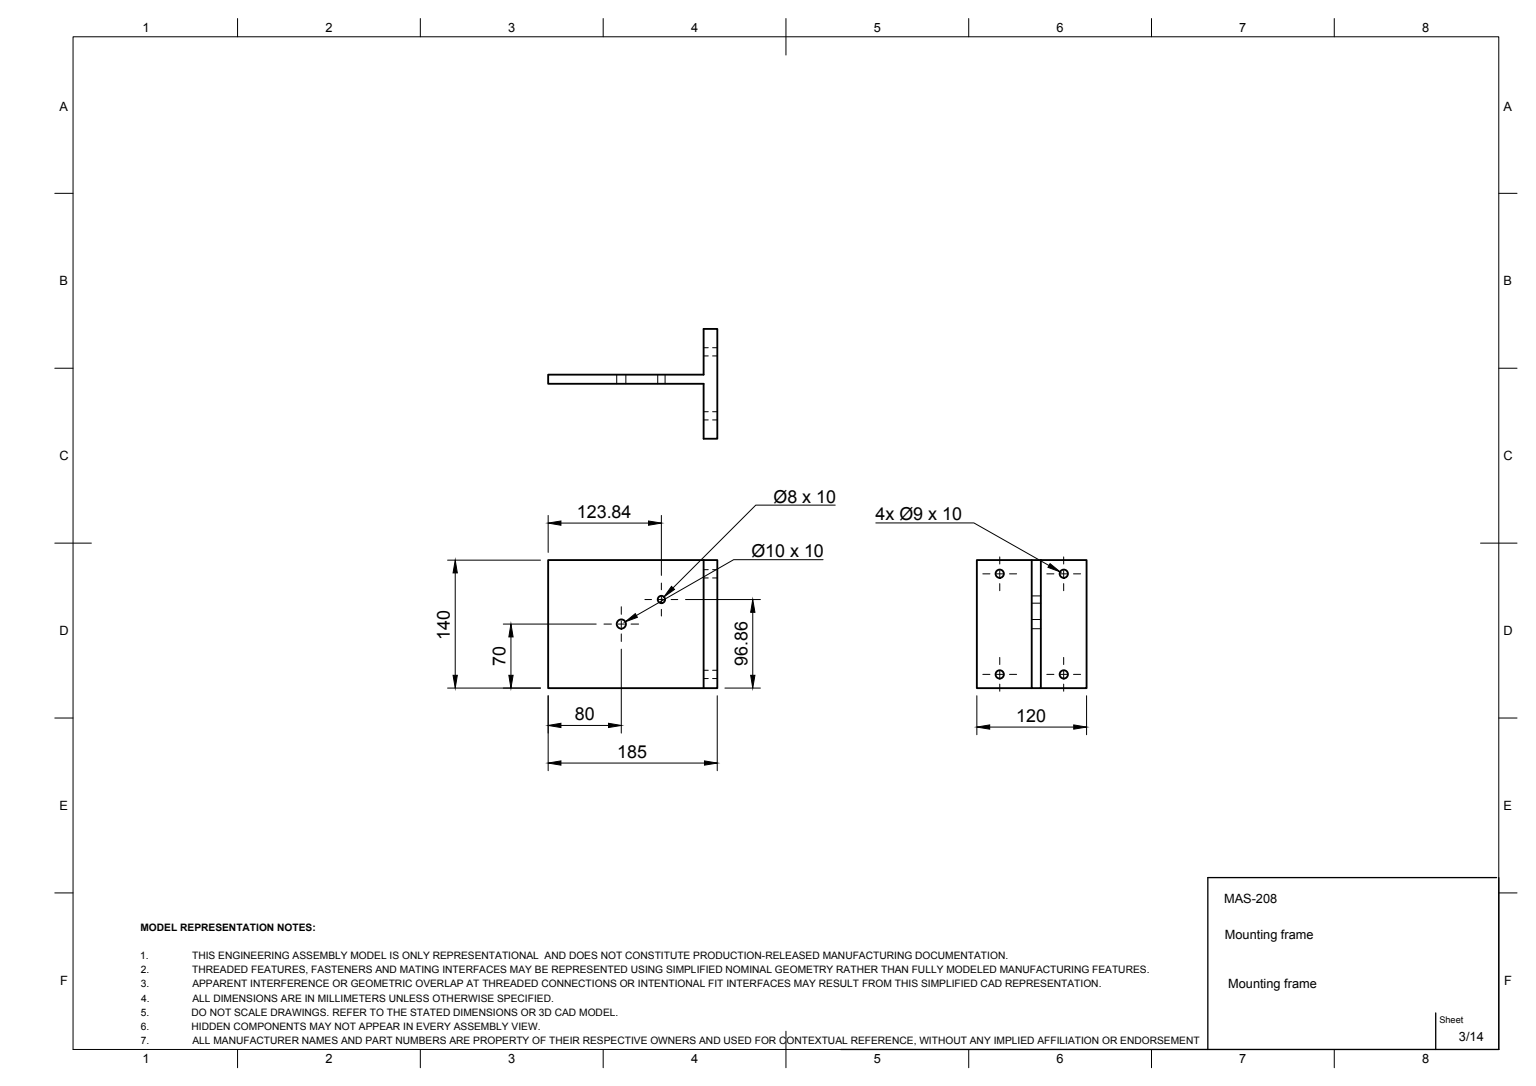
ISO-10303-21;
HEADER;
/* Generated by software containing ST-Developer
 * from STEP Tools, Inc. (www.steptools.com) 
 */

FILE_DESCRIPTION(
/* description */ ('Independent vertical20-tooth ratchet advance with repeated integral-c
ounterweight gravity pawls, swinging drive lever, bronze sleeves and f
ully retained axle stacks.18degpertooth. Native revolutes; geometric c
ycle checking rather than automatic contact/rolling dynamics. Gravity 
closing checked from actual pawl center of mass. Backplate/foot suppor
ts unit. Fits, torque, holding force, wear and life unassigned.'),
/* implementation_level */ '2;1');

FILE_NAME(
/* name */ 'Mounting frame.step',
/* time_stamp */ '2026-11-09T06:25:53-08:00',
/* author */ (''),
/* organization */ (''),
/* preprocessor_version */ 'ST-DEVELOPER v20.2',
/* originating_system */ 'Autodesk Translation Framework v15.17.0.0',
/* authorisation */ '');

FILE_SCHEMA (('AUTOMOTIVE_DESIGN { 1 0 10303 214 3 1 1 }'));
ENDSEC;

DATA;
#10=MECHANICAL_DESIGN_GEOMETRIC_PRESENTATION_REPRESENTATION('',(#123),#4643);
#95=SHAPE_REPRESENTATION_RELATIONSHIP('SRR','None',#4700,#109);
#109=ADVANCED_BREP_SHAPE_REPRESENTATION('',(#137),#4629);
#123=STYLED_ITEM('',(#4779),#137);
#137=MANIFOLD_SOLID_BREP('Body1',#2659);
#151=FACE_BOUND('',#460,.T.);
#152=FACE_BOUND('',#461,.T.);
#153=FACE_BOUND('',#463,.T.);
#154=FACE_BOUND('',#464,.T.);
#155=FACE_BOUND('',#466,.T.);
#156=FACE_BOUND('',#467,.T.);
#157=FACE_BOUND('',#468,.T.);
#158=FACE_BOUND('',#469,.T.);
#159=FACE_BOUND('',#476,.T.);
#160=FACE_BOUND('',#477,.T.);
#161=FACE_BOUND('',#479,.T.);
#162=FACE_BOUND('',#480,.T.);
#192=PLANE('',#2848);
#193=PLANE('',#2849);
#194=PLANE('',#2850);
#195=PLANE('',#2851);
#196=PLANE('',#2852);
#197=PLANE('',#2853);
#198=PLANE('',#2854);
#199=PLANE('',#2855);
#200=PLANE('',#2856);
#201=PLANE('',#2857);
#304=FACE_OUTER_BOUND('',#453,.T.);
#305=FACE_OUTER_BOUND('',#454,.T.);
#306=FACE_OUTER_BOUND('',#455,.T.);
#307=FACE_OUTER_BOUND('',#456,.T.);
#308=FACE_OUTER_BOUND('',#457,.T.);
#309=FACE_OUTER_BOUND('',#458,.T.);
#310=FACE_OUTER_BOUND('',#459,.T.);
#311=FACE_OUTER_BOUND('',#462,.T.);
#312=FACE_OUTER_BOUND('',#465,.T.);
#313=FACE_OUTER_BOUND('',#470,.T.);
#314=FACE_OUTER_BOUND('',#471,.T.);
#315=FACE_OUTER_BOUND('',#472,.T.);
#316=FACE_OUTER_BOUND('',#473,.T.);
#317=FACE_OUTER_BOUND('',#474,.T.);
#318=FACE_OUTER_BOUND('',#475,.T.);
#319=FACE_OUTER_BOUND('',#478,.T.);
#453=EDGE_LOOP('',(#1801,#1802,#1803,#1804));
#454=EDGE_LOOP('',(#1805,#1806,#1807,#1808));
#455=EDGE_LOOP('',(#1809,#1810,#1811,#1812));
#456=EDGE_LOOP('',(#1813,#1814,#1815,#1816));
#457=EDGE_LOOP('',(#1817,#1818,#1819,#1820));
#458=EDGE_LOOP('',(#1821,#1822,#1823,#1824));
#459=EDGE_LOOP('',(#1825,#1826,#1827,#1828));
#460=EDGE_LOOP('',(#1829));
#461=EDGE_LOOP('',(#1830));
#462=EDGE_LOOP('',(#1831,#1832,#1833,#1834));
#463=EDGE_LOOP('',(#1835));
#464=EDGE_LOOP('',(#1836));
#465=EDGE_LOOP('',(#1837,#1838,#1839,#1840));
#466=EDGE_LOOP('',(#1841));
#467=EDGE_LOOP('',(#1842));
#468=EDGE_LOOP('',(#1843));
#469=EDGE_LOOP('',(#1844));
#470=EDGE_LOOP('',(#1845,#1846,#1847,#1848));
#471=EDGE_LOOP('',(#1849,#1850,#1851,#1852));
#472=EDGE_LOOP('',(#1853,#1854,#1855,#1856));
#473=EDGE_LOOP('',(#1857,#1858,#1859,#1860,#1861,#1862,#1863,#1864));
#474=EDGE_LOOP('',(#1865,#1866,#1867,#1868,#1869,#1870,#1871,#1872));
#475=EDGE_LOOP('',(#1873,#1874,#1875,#1876));
#476=EDGE_LOOP('',(#1877));
#477=EDGE_LOOP('',(#1878));
#478=EDGE_LOOP('',(#1879,#1880,#1881,#1882));
#479=EDGE_LOOP('',(#1883));
#480=EDGE_LOOP('',(#1884));
#643=LINE('',#3873,#905);
#644=LINE('',#3879,#906);
#645=LINE('',#3885,#907);
#646=LINE('',#3891,#908);
#647=LINE('',#3897,#909);
#648=LINE('',#3903,#910);
#649=LINE('',#3908,#911);
#650=LINE('',#3910,#912);
#651=LINE('',#3912,#913);
#652=LINE('',#3913,#914);
#653=LINE('',#3917,#915);
#654=LINE('',#3919,#916);
#655=LINE('',#3921,#917);
#656=LINE('',#3922,#918);
#657=LINE('',#3926,#919);
#658=LINE('',#3928,#920);
#659=LINE('',#3930,#921);
#660=LINE('',#3931,#922);
#661=LINE('',#3933,#923);
#662=LINE('',#3934,#924);
#663=LINE('',#3936,#925);
#664=LINE('',#3937,#926);
#665=LINE('',#3941,#927);
#666=LINE('',#3943,#928);
#667=LINE('',#3945,#929);
#668=LINE('',#3946,#930);
#669=LINE('',#3948,#931);
#670=LINE('',#3949,#932);
#671=LINE('',#3951,#933);
#672=LINE('',#3952,#934);
#905=VECTOR('',#3095,4.);
#906=VECTOR('',#3102,5.);
#907=VECTOR('',#3109,4.5);
#908=VECTOR('',#3116,4.5);
#909=VECTOR('',#3123,4.5);
#910=VECTOR('',#3130,4.5);
#911=VECTOR('',#3135,10.);
#912=VECTOR('',#3136,10.);
#913=VECTOR('',#3137,10.);
#914=VECTOR('',#3138,10.);
#915=VECTOR('',#3141,10.);
#916=VECTOR('',#3142,10.);
#917=VECTOR('',#3143,10.);
#918=VECTOR('',#3144,10.);
#919=VECTOR('',#3147,10.);
#920=VECTOR('',#3148,10.);
#921=VECTOR('',#3149,10.);
#922=VECTOR('',#3150,10.);
#923=VECTOR('',#3153,10.);
#924=VECTOR('',#3154,10.);
#925=VECTOR('',#3157,10.);
#926=VECTOR('',#3158,10.);
#927=VECTOR('',#3161,10.);
#928=VECTOR('',#3162,10.);
#929=VECTOR('',#3163,10.);
#930=VECTOR('',#3164,10.);
#931=VECTOR('',#3167,10.);
#932=VECTOR('',#3168,10.);
#933=VECTOR('',#3171,10.);
#934=VECTOR('',#3172,10.);
#1167=CIRCLE('',#2831,4.);
#1168=CIRCLE('',#2832,4.);
#1169=CIRCLE('',#2834,5.);
#1170=CIRCLE('',#2835,5.);
#1171=CIRCLE('',#2837,4.5);
#1172=CIRCLE('',#2838,4.5);
#1173=CIRCLE('',#2840,4.5);
#1174=CIRCLE('',#2841,4.5);
#1175=CIRCLE('',#2843,4.5);
#1176=CIRCLE('',#2844,4.5);
#1177=CIRCLE('',#2846,4.5);
#1178=CIRCLE('',#2847,4.5);
#1241=VERTEX_POINT('',#3870);
#1242=VERTEX_POINT('',#3872);
#1243=VERTEX_POINT('',#3876);
#1244=VERTEX_POINT('',#3878);
#1245=VERTEX_POINT('',#3882);
#1246=VERTEX_POINT('',#3884);
#1247=VERTEX_POINT('',#3888);
#1248=VERTEX_POINT('',#3890);
#1249=VERTEX_POINT('',#3894);
#1250=VERTEX_POINT('',#3896);
#1251=VERTEX_POINT('',#3900);
#1252=VERTEX_POINT('',#3902);
#1253=VERTEX_POINT('',#3906);
#1254=VERTEX_POINT('',#3907);
#1255=VERTEX_POINT('',#3909);
#1256=VERTEX_POINT('',#3911);
#1257=VERTEX_POINT('',#3915);
#1258=VERTEX_POINT('',#3916);
#1259=VERTEX_POINT('',#3918);
#1260=VERTEX_POINT('',#3920);
#1261=VERTEX_POINT('',#3924);
#1262=VERTEX_POINT('',#3925);
#1263=VERTEX_POINT('',#3927);
#1264=VERTEX_POINT('',#3929);
#1265=VERTEX_POINT('',#3939);
#1266=VERTEX_POINT('',#3940);
#1267=VERTEX_POINT('',#3942);
#1268=VERTEX_POINT('',#3944);
#1465=EDGE_CURVE('',#1241,#1241,#1167,.T.);
#1466=EDGE_CURVE('',#1241,#1242,#643,.T.);
#1467=EDGE_CURVE('',#1242,#1242,#1168,.T.);
#1468=EDGE_CURVE('',#1243,#1243,#1169,.T.);
#1469=EDGE_CURVE('',#1243,#1244,#644,.T.);
#1470=EDGE_CURVE('',#1244,#1244,#1170,.T.);
#1471=EDGE_CURVE('',#1245,#1245,#1171,.F.);
#1472=EDGE_CURVE('',#1245,#1246,#645,.T.);
#1473=EDGE_CURVE('',#1246,#1246,#1172,.T.);
#1474=EDGE_CURVE('',#1247,#1247,#1173,.F.);
#1475=EDGE_CURVE('',#1247,#1248,#646,.T.);
#1476=EDGE_CURVE('',#1248,#1248,#1174,.T.);
#1477=EDGE_CURVE('',#1249,#1249,#1175,.F.);
#1478=EDGE_CURVE('',#1249,#1250,#647,.T.);
#1479=EDGE_CURVE('',#1250,#1250,#1176,.T.);
#1480=EDGE_CURVE('',#1251,#1251,#1177,.F.);
#1481=EDGE_CURVE('',#1251,#1252,#648,.T.);
#1482=EDGE_CURVE('',#1252,#1252,#1178,.T.);
#1483=EDGE_CURVE('',#1253,#1254,#649,.T.);
#1484=EDGE_CURVE('',#1255,#1254,#650,.T.);
#1485=EDGE_CURVE('',#1255,#1256,#651,.T.);
#1486=EDGE_CURVE('',#1256,#1253,#652,.T.);
#1487=EDGE_CURVE('',#1257,#1258,#653,.T.);
#1488=EDGE_CURVE('',#1257,#1259,#654,.T.);
#1489=EDGE_CURVE('',#1260,#1259,#655,.T.);
#1490=EDGE_CURVE('',#1258,#1260,#656,.T.);
#1491=EDGE_CURVE('',#1261,#1262,#657,.T.);
#1492=EDGE_CURVE('',#1262,#1263,#658,.T.);
#1493=EDGE_CURVE('',#1264,#1263,#659,.F.);
#1494=EDGE_CURVE('',#1261,#1264,#660,.F.);
#1495=EDGE_CURVE('',#1259,#1264,#661,.T.);
#1496=EDGE_CURVE('',#1263,#1260,#662,.T.);
#1497=EDGE_CURVE('',#1256,#1261,#663,.T.);
#1498=EDGE_CURVE('',#1262,#1255,#664,.T.);
#1499=EDGE_CURVE('',#1265,#1266,#665,.F.);
#1500=EDGE_CURVE('',#1266,#1267,#666,.T.);
#1501=EDGE_CURVE('',#1268,#1267,#667,.F.);
#1502=EDGE_CURVE('',#1265,#1268,#668,.F.);
#1503=EDGE_CURVE('',#1254,#1265,#669,.T.);
#1504=EDGE_CURVE('',#1258,#1268,#670,.T.);
#1505=EDGE_CURVE('',#1266,#1253,#671,.T.);
#1506=EDGE_CURVE('',#1267,#1257,#672,.T.);
#1801=ORIENTED_EDGE('',*,*,#1465,.F.);
#1802=ORIENTED_EDGE('',*,*,#1466,.T.);
#1803=ORIENTED_EDGE('',*,*,#1467,.F.);
#1804=ORIENTED_EDGE('',*,*,#1466,.F.);
#1805=ORIENTED_EDGE('',*,*,#1468,.F.);
#1806=ORIENTED_EDGE('',*,*,#1469,.T.);
#1807=ORIENTED_EDGE('',*,*,#1470,.F.);
#1808=ORIENTED_EDGE('',*,*,#1469,.F.);
#1809=ORIENTED_EDGE('',*,*,#1471,.F.);
#1810=ORIENTED_EDGE('',*,*,#1472,.T.);
#1811=ORIENTED_EDGE('',*,*,#1473,.F.);
#1812=ORIENTED_EDGE('',*,*,#1472,.F.);
#1813=ORIENTED_EDGE('',*,*,#1474,.F.);
#1814=ORIENTED_EDGE('',*,*,#1475,.T.);
#1815=ORIENTED_EDGE('',*,*,#1476,.F.);
#1816=ORIENTED_EDGE('',*,*,#1475,.F.);
#1817=ORIENTED_EDGE('',*,*,#1477,.F.);
#1818=ORIENTED_EDGE('',*,*,#1478,.T.);
#1819=ORIENTED_EDGE('',*,*,#1479,.F.);
#1820=ORIENTED_EDGE('',*,*,#1478,.F.);
#1821=ORIENTED_EDGE('',*,*,#1480,.F.);
#1822=ORIENTED_EDGE('',*,*,#1481,.T.);
#1823=ORIENTED_EDGE('',*,*,#1482,.F.);
#1824=ORIENTED_EDGE('',*,*,#1481,.F.);
#1825=ORIENTED_EDGE('',*,*,#1483,.T.);
#1826=ORIENTED_EDGE('',*,*,#1484,.F.);
#1827=ORIENTED_EDGE('',*,*,#1485,.T.);
#1828=ORIENTED_EDGE('',*,*,#1486,.T.);
#1829=ORIENTED_EDGE('',*,*,#1473,.T.);
#1830=ORIENTED_EDGE('',*,*,#1476,.T.);
#1831=ORIENTED_EDGE('',*,*,#1487,.F.);
#1832=ORIENTED_EDGE('',*,*,#1488,.T.);
#1833=ORIENTED_EDGE('',*,*,#1489,.F.);
#1834=ORIENTED_EDGE('',*,*,#1490,.F.);
#1835=ORIENTED_EDGE('',*,*,#1479,.T.);
#1836=ORIENTED_EDGE('',*,*,#1482,.T.);
#1837=ORIENTED_EDGE('',*,*,#1491,.T.);
#1838=ORIENTED_EDGE('',*,*,#1492,.T.);
#1839=ORIENTED_EDGE('',*,*,#1493,.F.);
#1840=ORIENTED_EDGE('',*,*,#1494,.F.);
#1841=ORIENTED_EDGE('',*,*,#1471,.T.);
#1842=ORIENTED_EDGE('',*,*,#1474,.T.);
#1843=ORIENTED_EDGE('',*,*,#1477,.T.);
#1844=ORIENTED_EDGE('',*,*,#1480,.T.);
#1845=ORIENTED_EDGE('',*,*,#1495,.T.);
#1846=ORIENTED_EDGE('',*,*,#1493,.T.);
#1847=ORIENTED_EDGE('',*,*,#1496,.T.);
#1848=ORIENTED_EDGE('',*,*,#1489,.T.);
#1849=ORIENTED_EDGE('',*,*,#1497,.F.);
#1850=ORIENTED_EDGE('',*,*,#1485,.F.);
#1851=ORIENTED_EDGE('',*,*,#1498,.F.);
#1852=ORIENTED_EDGE('',*,*,#1491,.F.);
#1853=ORIENTED_EDGE('',*,*,#1499,.T.);
#1854=ORIENTED_EDGE('',*,*,#1500,.T.);
#1855=ORIENTED_EDGE('',*,*,#1501,.F.);
#1856=ORIENTED_EDGE('',*,*,#1502,.F.);
#1857=ORIENTED_EDGE('',*,*,#1503,.T.);
#1858=ORIENTED_EDGE('',*,*,#1502,.T.);
#1859=ORIENTED_EDGE('',*,*,#1504,.F.);
#1860=ORIENTED_EDGE('',*,*,#1490,.T.);
#1861=ORIENTED_EDGE('',*,*,#1496,.F.);
#1862=ORIENTED_EDGE('',*,*,#1492,.F.);
#1863=ORIENTED_EDGE('',*,*,#1498,.T.);
#1864=ORIENTED_EDGE('',*,*,#1484,.T.);
#1865=ORIENTED_EDGE('',*,*,#1505,.T.);
#1866=ORIENTED_EDGE('',*,*,#1486,.F.);
#1867=ORIENTED_EDGE('',*,*,#1497,.T.);
#1868=ORIENTED_EDGE('',*,*,#1494,.T.);
#1869=ORIENTED_EDGE('',*,*,#1495,.F.);
#1870=ORIENTED_EDGE('',*,*,#1488,.F.);
#1871=ORIENTED_EDGE('',*,*,#1506,.F.);
#1872=ORIENTED_EDGE('',*,*,#1500,.F.);
#1873=ORIENTED_EDGE('',*,*,#1506,.T.);
#1874=ORIENTED_EDGE('',*,*,#1487,.T.);
#1875=ORIENTED_EDGE('',*,*,#1504,.T.);
#1876=ORIENTED_EDGE('',*,*,#1501,.T.);
#1877=ORIENTED_EDGE('',*,*,#1465,.T.);
#1878=ORIENTED_EDGE('',*,*,#1468,.T.);
#1879=ORIENTED_EDGE('',*,*,#1505,.F.);
#1880=ORIENTED_EDGE('',*,*,#1499,.F.);
#1881=ORIENTED_EDGE('',*,*,#1503,.F.);
#1882=ORIENTED_EDGE('',*,*,#1483,.F.);
#1883=ORIENTED_EDGE('',*,*,#1467,.T.);
#1884=ORIENTED_EDGE('',*,*,#1470,.T.);
#2473=CYLINDRICAL_SURFACE('',#2830,4.);
#2474=CYLINDRICAL_SURFACE('',#2833,5.);
#2475=CYLINDRICAL_SURFACE('',#2836,4.5);
#2476=CYLINDRICAL_SURFACE('',#2839,4.5);
#2477=CYLINDRICAL_SURFACE('',#2842,4.5);
#2478=CYLINDRICAL_SURFACE('',#2845,4.5);
#2510=ADVANCED_FACE('',(#304),#2473,.F.);
#2511=ADVANCED_FACE('',(#305),#2474,.F.);
#2512=ADVANCED_FACE('',(#306),#2475,.F.);
#2513=ADVANCED_FACE('',(#307),#2476,.F.);
#2514=ADVANCED_FACE('',(#308),#2477,.F.);
#2515=ADVANCED_FACE('',(#309),#2478,.F.);
#2516=ADVANCED_FACE('',(#310,#151,#152),#192,.T.);
#2517=ADVANCED_FACE('',(#311,#153,#154),#193,.T.);
#2518=ADVANCED_FACE('',(#312,#155,#156,#157,#158),#194,.T.);
#2519=ADVANCED_FACE('',(#313),#195,.T.);
#2520=ADVANCED_FACE('',(#314),#196,.F.);
#2521=ADVANCED_FACE('',(#315),#197,.T.);
#2522=ADVANCED_FACE('',(#316),#198,.T.);
#2523=ADVANCED_FACE('',(#317),#199,.T.);
#2524=ADVANCED_FACE('',(#318,#159,#160),#200,.T.);
#2525=ADVANCED_FACE('',(#319,#161,#162),#201,.F.);
#2659=CLOSED_SHELL('',(#2510,#2511,#2512,#2513,#2514,#2515,#2516,#2517,
#2518,#2519,#2520,#2521,#2522,#2523,#2524,#2525));
#2829=AXIS2_PLACEMENT_3D('',#3868,#3089,#3090);
#2830=AXIS2_PLACEMENT_3D('',#3869,#3091,#3092);
#2831=AXIS2_PLACEMENT_3D('',#3871,#3093,#3094);
#2832=AXIS2_PLACEMENT_3D('',#3874,#3096,#3097);
#2833=AXIS2_PLACEMENT_3D('',#3875,#3098,#3099);
#2834=AXIS2_PLACEMENT_3D('',#3877,#3100,#3101);
#2835=AXIS2_PLACEMENT_3D('',#3880,#3103,#3104);
#2836=AXIS2_PLACEMENT_3D('',#3881,#3105,#3106);
#2837=AXIS2_PLACEMENT_3D('',#3883,#3107,#3108);
#2838=AXIS2_PLACEMENT_3D('',#3886,#3110,#3111);
#2839=AXIS2_PLACEMENT_3D('',#3887,#3112,#3113);
#2840=AXIS2_PLACEMENT_3D('',#3889,#3114,#3115);
#2841=AXIS2_PLACEMENT_3D('',#3892,#3117,#3118);
#2842=AXIS2_PLACEMENT_3D('',#3893,#3119,#3120);
#2843=AXIS2_PLACEMENT_3D('',#3895,#3121,#3122);
#2844=AXIS2_PLACEMENT_3D('',#3898,#3124,#3125);
#2845=AXIS2_PLACEMENT_3D('',#3899,#3126,#3127);
#2846=AXIS2_PLACEMENT_3D('',#3901,#3128,#3129);
#2847=AXIS2_PLACEMENT_3D('',#3904,#3131,#3132);
#2848=AXIS2_PLACEMENT_3D('',#3905,#3133,#3134);
#2849=AXIS2_PLACEMENT_3D('',#3914,#3139,#3140);
#2850=AXIS2_PLACEMENT_3D('',#3923,#3145,#3146);
#2851=AXIS2_PLACEMENT_3D('',#3932,#3151,#3152);
#2852=AXIS2_PLACEMENT_3D('',#3935,#3155,#3156);
#2853=AXIS2_PLACEMENT_3D('',#3938,#3159,#3160);
#2854=AXIS2_PLACEMENT_3D('',#3947,#3165,#3166);
#2855=AXIS2_PLACEMENT_3D('',#3950,#3169,#3170);
#2856=AXIS2_PLACEMENT_3D('',#3953,#3173,#3174);
#2857=AXIS2_PLACEMENT_3D('',#3954,#3175,#3176);
#3089=DIRECTION('axis',(0.,0.,1.));
#3090=DIRECTION('refdir',(1.,0.,0.));
#3091=DIRECTION('center_axis',(0.,0.,-1.));
#3092=DIRECTION('ref_axis',(1.,0.,0.));
#3093=DIRECTION('center_axis',(0.,0.,-1.));
#3094=DIRECTION('ref_axis',(1.,0.,0.));
#3095=DIRECTION('',(0.,0.,-1.));
#3096=DIRECTION('center_axis',(0.,0.,1.));
#3097=DIRECTION('ref_axis',(1.,0.,0.));
#3098=DIRECTION('center_axis',(0.,0.,-1.));
#3099=DIRECTION('ref_axis',(1.,0.,0.));
#3100=DIRECTION('center_axis',(0.,0.,-1.));
#3101=DIRECTION('ref_axis',(1.,0.,0.));
#3102=DIRECTION('',(0.,0.,-1.));
#3103=DIRECTION('center_axis',(0.,0.,1.));
#3104=DIRECTION('ref_axis',(1.,0.,0.));
#3105=DIRECTION('center_axis',(0.,1.,0.));
#3106=DIRECTION('ref_axis',(0.,0.,-1.));
#3107=DIRECTION('center_axis',(0.,-1.,0.));
#3108=DIRECTION('ref_axis',(0.,0.,-1.));
#3109=DIRECTION('',(0.,1.,0.));
#3110=DIRECTION('center_axis',(0.,-1.,0.));
#3111=DIRECTION('ref_axis',(0.,0.,-1.));
#3112=DIRECTION('center_axis',(0.,1.,0.));
#3113=DIRECTION('ref_axis',(0.,0.,-1.));
#3114=DIRECTION('center_axis',(0.,-1.,0.));
#3115=DIRECTION('ref_axis',(0.,0.,-1.));
#3116=DIRECTION('',(0.,1.,0.));
#3117=DIRECTION('center_axis',(0.,-1.,0.));
#3118=DIRECTION('ref_axis',(0.,0.,-1.));
#3119=DIRECTION('center_axis',(0.,1.,0.));
#3120=DIRECTION('ref_axis',(0.,0.,-1.));
#3121=DIRECTION('center_axis',(0.,-1.,0.));
#3122=DIRECTION('ref_axis',(0.,0.,-1.));
#3123=DIRECTION('',(0.,1.,0.));
#3124=DIRECTION('center_axis',(0.,-1.,0.));
#3125=DIRECTION('ref_axis',(0.,0.,-1.));
#3126=DIRECTION('center_axis',(0.,1.,0.));
#3127=DIRECTION('ref_axis',(0.,0.,-1.));
#3128=DIRECTION('center_axis',(0.,-1.,0.));
#3129=DIRECTION('ref_axis',(0.,0.,-1.));
#3130=DIRECTION('',(0.,1.,0.));
#3131=DIRECTION('center_axis',(0.,-1.,0.));
#3132=DIRECTION('ref_axis',(0.,0.,-1.));
#3133=DIRECTION('center_axis',(0.,1.,0.));
#3134=DIRECTION('ref_axis',(-1.,0.,0.));
#3135=DIRECTION('',(1.,0.,0.));
#3136=DIRECTION('',(0.,0.,1.));
#3137=DIRECTION('',(-1.,0.,0.));
#3138=DIRECTION('',(0.,0.,1.));
#3139=DIRECTION('center_axis',(0.,1.,0.));
#3140=DIRECTION('ref_axis',(-1.,0.,0.));
#3141=DIRECTION('',(1.,0.,0.));
#3142=DIRECTION('',(0.,0.,1.));
#3143=DIRECTION('',(-1.,0.,0.));
#3144=DIRECTION('',(0.,0.,1.));
#3145=DIRECTION('center_axis',(0.,-1.,0.));
#3146=DIRECTION('ref_axis',(1.,0.,0.));
#3147=DIRECTION('',(1.,0.,0.));
#3148=DIRECTION('',(0.,0.,1.));
#3149=DIRECTION('',(-1.,0.,0.));
#3150=DIRECTION('',(0.,0.,-1.));
#3151=DIRECTION('center_axis',(0.,0.,1.));
#3152=DIRECTION('ref_axis',(1.,0.,0.));
#3153=DIRECTION('',(0.,-1.,0.));
#3154=DIRECTION('',(0.,1.,0.));
#3155=DIRECTION('center_axis',(0.,0.,1.));
#3156=DIRECTION('ref_axis',(1.,0.,0.));
#3157=DIRECTION('',(0.,-1.,0.));
#3158=DIRECTION('',(0.,1.,0.));
#3159=DIRECTION('center_axis',(0.,1.,0.));
#3160=DIRECTION('ref_axis',(-1.,0.,0.));
#3161=DIRECTION('',(1.,0.,0.));
#3162=DIRECTION('',(0.,0.,1.));
#3163=DIRECTION('',(1.,0.,0.));
#3164=DIRECTION('',(0.,0.,-1.));
#3165=DIRECTION('center_axis',(1.,0.,0.));
#3166=DIRECTION('ref_axis',(0.,1.,0.));
#3167=DIRECTION('',(0.,1.,0.));
#3168=DIRECTION('',(0.,1.,0.));
#3169=DIRECTION('center_axis',(-1.,0.,0.));
#3170=DIRECTION('ref_axis',(0.,-1.,0.));
#3171=DIRECTION('',(0.,-1.,0.));
#3172=DIRECTION('',(0.,-1.,0.));
#3173=DIRECTION('center_axis',(0.,0.,1.));
#3174=DIRECTION('ref_axis',(1.,0.,0.));
#3175=DIRECTION('center_axis',(0.,0.,1.));
#3176=DIRECTION('ref_axis',(1.,0.,0.));
#3868=CARTESIAN_POINT('',(0.,0.,0.));
#3869=CARTESIAN_POINT('Origin',(26.8635279142892,-43.8446218822583,5.));
#3870=CARTESIAN_POINT('',(22.8635279142892,-43.8446218822583,10.));
#3871=CARTESIAN_POINT('Origin',(26.8635279142892,-43.8446218822583,10.));
#3872=CARTESIAN_POINT('',(22.8635279142892,-43.8446218822583,0.));
#3873=CARTESIAN_POINT('',(22.8635279142892,-43.8446218822583,5.));
#3874=CARTESIAN_POINT('Origin',(26.8635279142892,-43.8446218822583,0.));
#3875=CARTESIAN_POINT('Origin',(0.,0.,5.));
#3876=CARTESIAN_POINT('',(-5.,6.12323399573677E-16,10.));
#3877=CARTESIAN_POINT('Origin',(0.,0.,10.));
#3878=CARTESIAN_POINT('',(-5.,6.12323399573677E-16,0.));
#3879=CARTESIAN_POINT('',(-5.,6.12323399573677E-16,5.));
#3880=CARTESIAN_POINT('Origin',(0.,0.,0.));
#3881=CARTESIAN_POINT('Origin',(55.,-95.,-35.));
#3882=CARTESIAN_POINT('',(55.,-105.,-30.5));
#3883=CARTESIAN_POINT('Origin',(55.,-105.,-35.));
#3884=CARTESIAN_POINT('',(55.,-90.,-30.5));
#3885=CARTESIAN_POINT('',(55.,-95.,-30.5));
#3886=CARTESIAN_POINT('Origin',(55.,-90.,-35.));
#3887=CARTESIAN_POINT('Origin',(-55.,-95.,-35.));
#3888=CARTESIAN_POINT('',(-55.,-105.,-30.5));
#3889=CARTESIAN_POINT('Origin',(-55.,-105.,-35.));
#3890=CARTESIAN_POINT('',(-55.,-90.,-30.5));
#3891=CARTESIAN_POINT('',(-55.,-95.,-30.5));
#3892=CARTESIAN_POINT('Origin',(-55.,-90.,-35.));
#3893=CARTESIAN_POINT('Origin',(-55.,-95.,35.));
#3894=CARTESIAN_POINT('',(-55.,-105.,39.5));
#3895=CARTESIAN_POINT('Origin',(-55.,-105.,35.));
#3896=CARTESIAN_POINT('',(-55.,-90.,39.5));
#3897=CARTESIAN_POINT('',(-55.,-95.,39.5));
#3898=CARTESIAN_POINT('Origin',(-55.,-90.,35.));
#3899=CARTESIAN_POINT('Origin',(55.,-95.,35.));
#3900=CARTESIAN_POINT('',(55.,-105.,39.5));
#3901=CARTESIAN_POINT('Origin',(55.,-105.,35.));
#3902=CARTESIAN_POINT('',(55.,-90.,39.5));
#3903=CARTESIAN_POINT('',(55.,-95.,39.5));
#3904=CARTESIAN_POINT('Origin',(55.,-90.,35.));
#3905=CARTESIAN_POINT('Origin',(70.,-90.,-40.));
#3906=CARTESIAN_POINT('',(-70.,-90.,0.));
#3907=CARTESIAN_POINT('',(70.,-90.,0.));
#3908=CARTESIAN_POINT('',(-70.,-90.,0.));
#3909=CARTESIAN_POINT('',(70.,-90.,-60.));
#3910=CARTESIAN_POINT('',(70.,-90.,-40.));
#3911=CARTESIAN_POINT('',(-70.,-90.,-60.));
#3912=CARTESIAN_POINT('',(35.,-90.,-60.));
#3913=CARTESIAN_POINT('',(-70.,-90.,-40.));
#3914=CARTESIAN_POINT('Origin',(70.,-90.,-40.));
#3915=CARTESIAN_POINT('',(-70.,-90.,10.));
#3916=CARTESIAN_POINT('',(70.,-90.,10.));
#3917=CARTESIAN_POINT('',(-70.,-90.,10.));
#3918=CARTESIAN_POINT('',(-70.,-90.,60.));
#3919=CARTESIAN_POINT('',(-70.,-90.,-40.));
#3920=CARTESIAN_POINT('',(70.,-90.,60.));
#3921=CARTESIAN_POINT('',(70.,-90.,60.));
#3922=CARTESIAN_POINT('',(70.,-90.,-40.));
#3923=CARTESIAN_POINT('Origin',(-70.,-105.,-40.));
#3924=CARTESIAN_POINT('',(-70.,-105.,-60.));
#3925=CARTESIAN_POINT('',(70.,-105.,-60.));
#3926=CARTESIAN_POINT('',(-35.,-105.,-60.));
#3927=CARTESIAN_POINT('',(70.,-105.,60.));
#3928=CARTESIAN_POINT('',(70.,-105.,-20.));
#3929=CARTESIAN_POINT('',(-70.,-105.,60.));
#3930=CARTESIAN_POINT('',(-35.,-105.,60.));
#3931=CARTESIAN_POINT('',(-70.,-105.,-20.));
#3932=CARTESIAN_POINT('Origin',(0.,-95.,60.));
#3933=CARTESIAN_POINT('',(-70.,-90.,60.));
#3934=CARTESIAN_POINT('',(70.,-100.,60.));
#3935=CARTESIAN_POINT('Origin',(0.,-95.,-60.));
#3936=CARTESIAN_POINT('',(-70.,-2.5,-60.));
#3937=CARTESIAN_POINT('',(70.,-92.5,-60.));
#3938=CARTESIAN_POINT('Origin',(70.,80.,0.));
#3939=CARTESIAN_POINT('',(70.,80.,0.));
#3940=CARTESIAN_POINT('',(-70.,80.,0.));
#3941=CARTESIAN_POINT('',(35.,80.,0.));
#3942=CARTESIAN_POINT('',(-70.,80.,10.));
#3943=CARTESIAN_POINT('',(-70.,80.,0.));
#3944=CARTESIAN_POINT('',(70.,80.,10.));
#3945=CARTESIAN_POINT('',(35.,80.,10.));
#3946=CARTESIAN_POINT('',(70.,80.,0.));
#3947=CARTESIAN_POINT('Origin',(70.,-90.,0.));
#3948=CARTESIAN_POINT('',(70.,-90.,0.));
#3949=CARTESIAN_POINT('',(70.,-90.,10.));
#3950=CARTESIAN_POINT('Origin',(-70.,90.,0.));
#3951=CARTESIAN_POINT('',(-70.,90.,0.));
#3952=CARTESIAN_POINT('',(-70.,90.,10.));
#3953=CARTESIAN_POINT('Origin',(0.,0.,10.));
#3954=CARTESIAN_POINT('Origin',(0.,0.,0.));
#4613=UNCERTAINTY_MEASURE_WITH_UNIT(LENGTH_MEASURE(0.01),#4644,
'DISTANCE_ACCURACY_VALUE',
'Maximum model space distance between geometric entities at asserted c
onnectivities');
#4627=UNCERTAINTY_MEASURE_WITH_UNIT(LENGTH_MEASURE(0.01),#4644,
'DISTANCE_ACCURACY_VALUE',
'Maximum model space distance between geometric entities at asserted c
onnectivities');
#4629=(
GEOMETRIC_REPRESENTATION_CONTEXT(3)
GLOBAL_UNCERTAINTY_ASSIGNED_CONTEXT((#4613))
GLOBAL_UNIT_ASSIGNED_CONTEXT((#4644,#4646,#4647))
REPRESENTATION_CONTEXT('','3D')
);
#4643=(
GEOMETRIC_REPRESENTATION_CONTEXT(3)
GLOBAL_UNCERTAINTY_ASSIGNED_CONTEXT((#4627))
GLOBAL_UNIT_ASSIGNED_CONTEXT((#4644,#4646,#4647))
REPRESENTATION_CONTEXT('','3D')
);
#4644=(
LENGTH_UNIT()
NAMED_UNIT(*)
SI_UNIT(.MILLI.,.METRE.)
);
#4646=(
NAMED_UNIT(*)
PLANE_ANGLE_UNIT()
SI_UNIT($,.RADIAN.)
);
#4647=(
NAMED_UNIT(*)
SI_UNIT($,.STERADIAN.)
SOLID_ANGLE_UNIT()
);
#4649=SHAPE_DEFINITION_REPRESENTATION(#4664,#4700);
#4664=PRODUCT_DEFINITION_SHAPE('',$,#4716);
#4700=SHAPE_REPRESENTATION('',(#2829),#4629);
#4714=PRODUCT_DEFINITION_CONTEXT('part definition',#4761,'design');
#4716=PRODUCT_DEFINITION('Mounting frame','Mounting frame',#4731,#4714);
#4731=PRODUCT_DEFINITION_FORMATION('',$,#4764);
#4761=APPLICATION_CONTEXT(
'Core Data for Automotive Mechanical Design Process');
#4762=PRODUCT_CONTEXT('part definition',#4761,'mechanical');
#4764=PRODUCT('Mounting frame','Mounting frame',$,(#4762));
#4779=PRESENTATION_STYLE_ASSIGNMENT((#4788));
#4788=SURFACE_STYLE_USAGE(.BOTH.,#4797);
#4797=SURFACE_SIDE_STYLE('',(#4806));
#4806=SURFACE_STYLE_FILL_AREA(#4815);
#4815=FILL_AREA_STYLE('Frame gray',(#4824));
#4824=FILL_AREA_STYLE_COLOUR('Frame gray',#4833);
#4833=COLOUR_RGB('Frame gray',0.407843137254902,0.447058823529412,0.498039215686275);
ENDSEC;
END-ISO-10303-21;
